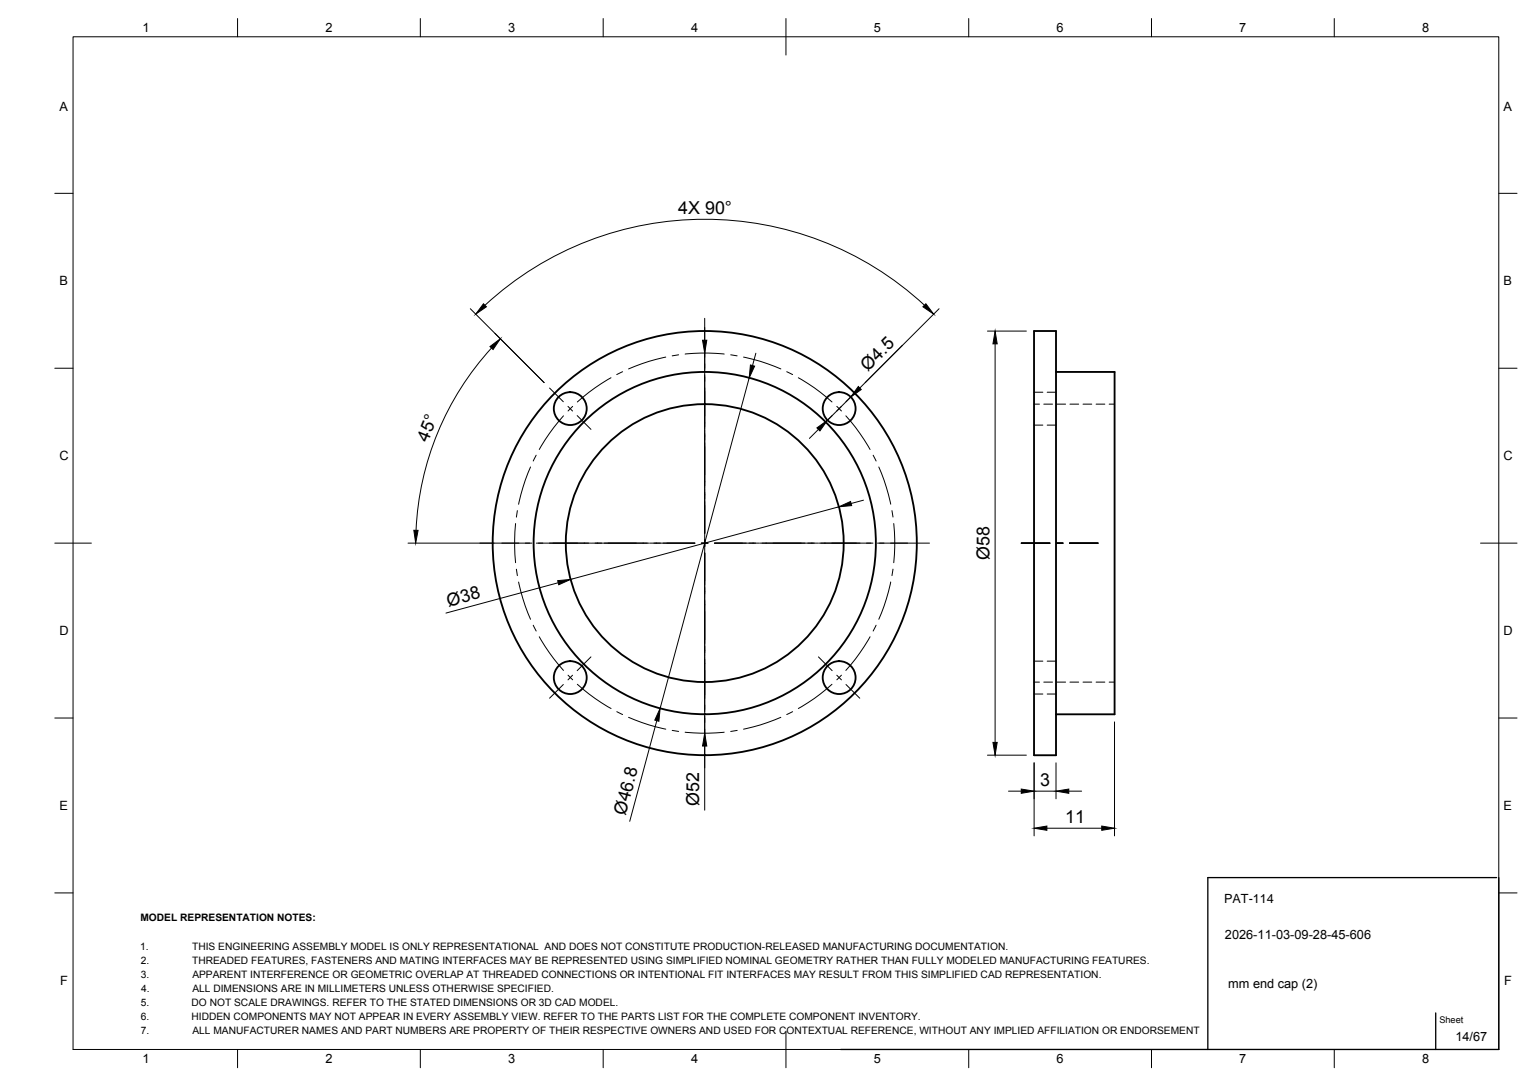
ISO-10303-21;
HEADER;
/* Generated by software containing ST-Developer
 * from STEP Tools, Inc. (www.steptools.com) 
 */

FILE_DESCRIPTION(
/* description */ ('Two-stage gear reducer in split housing'),
/* implementation_level */ '2;1');

FILE_NAME(
/* name */ 'mm end cap (2).step',
/* time_stamp */ '2026-10-28T03:22:31-07:00',
/* author */ (''),
/* organization */ (''),
/* preprocessor_version */ 'ST-DEVELOPER v20.2',
/* originating_system */ 'Autodesk Translation Framework v15.17.0.0',
/* authorisation */ '');

FILE_SCHEMA (('AUTOMOTIVE_DESIGN { 1 0 10303 214 3 1 1 }'));
ENDSEC;

DATA;
#10=MECHANICAL_DESIGN_GEOMETRIC_PRESENTATION_REPRESENTATION('',(#1243),#73366);
#1131=SHAPE_REPRESENTATION_RELATIONSHIP('SRR','None',#73618,#1187);
#1187=ADVANCED_BREP_SHAPE_REPRESENTATION('',(#1314),#73314);
#1243=STYLED_ITEM('',(#74002),#1314);
#1314=MANIFOLD_SOLID_BREP('Body1',#16131);
#1466=FACE_BOUND('',#3233,.T.);
#1467=FACE_BOUND('',#3237,.T.);
#1468=FACE_BOUND('',#3238,.T.);
#1469=FACE_BOUND('',#3239,.T.);
#1470=FACE_BOUND('',#3240,.T.);
#1471=FACE_BOUND('',#3241,.T.);
#1472=FACE_BOUND('',#3243,.T.);
#1473=FACE_BOUND('',#3244,.T.);
#1474=FACE_BOUND('',#3245,.T.);
#1475=FACE_BOUND('',#3246,.T.);
#1476=FACE_BOUND('',#3247,.T.);
#1714=PLANE('',#17275);
#1715=PLANE('',#17282);
#1716=PLANE('',#17283);
#2222=FACE_OUTER_BOUND('',#3227,.T.);
#2223=FACE_OUTER_BOUND('',#3228,.T.);
#2224=FACE_OUTER_BOUND('',#3229,.T.);
#2225=FACE_OUTER_BOUND('',#3230,.T.);
#2226=FACE_OUTER_BOUND('',#3231,.T.);
#2227=FACE_OUTER_BOUND('',#3232,.T.);
#2228=FACE_OUTER_BOUND('',#3234,.T.);
#2229=FACE_OUTER_BOUND('',#3235,.T.);
#2230=FACE_OUTER_BOUND('',#3236,.T.);
#2231=FACE_OUTER_BOUND('',#3242,.T.);
#3227=EDGE_LOOP('',(#11491,#11492,#11493,#11494));
#3228=EDGE_LOOP('',(#11495,#11496,#11497,#11498));
#3229=EDGE_LOOP('',(#11499,#11500,#11501,#11502));
#3230=EDGE_LOOP('',(#11503,#11504,#11505,#11506));
#3231=EDGE_LOOP('',(#11507,#11508,#11509,#11510));
#3232=EDGE_LOOP('',(#11511));
#3233=EDGE_LOOP('',(#11512));
#3234=EDGE_LOOP('',(#11513,#11514,#11515,#11516));
#3235=EDGE_LOOP('',(#11517,#11518,#11519,#11520));
#3236=EDGE_LOOP('',(#11521));
#3237=EDGE_LOOP('',(#11522));
#3238=EDGE_LOOP('',(#11523));
#3239=EDGE_LOOP('',(#11524));
#3240=EDGE_LOOP('',(#11525));
#3241=EDGE_LOOP('',(#11526));
#3242=EDGE_LOOP('',(#11527));
#3243=EDGE_LOOP('',(#11528));
#3244=EDGE_LOOP('',(#11529));
#3245=EDGE_LOOP('',(#11530));
#3246=EDGE_LOOP('',(#11531));
#3247=EDGE_LOOP('',(#11532));
#4332=LINE('',#23830,#5356);
#4333=LINE('',#23836,#5357);
#4334=LINE('',#23842,#5358);
#4335=LINE('',#23848,#5359);
#4336=LINE('',#23854,#5360);
#4337=LINE('',#23861,#5361);
#4338=LINE('',#23867,#5362);
#5356=VECTOR('',#19634,0.225);
#5357=VECTOR('',#19641,0.225);
#5358=VECTOR('',#19648,0.225000000000001);
#5359=VECTOR('',#19655,0.225000000000001);
#5360=VECTOR('',#19662,2.34);
#5361=VECTOR('',#19671,1.9);
#5362=VECTOR('',#19678,2.9);
#6320=CIRCLE('',#17261,0.225);
#6321=CIRCLE('',#17262,0.225);
#6322=CIRCLE('',#17264,0.225);
#6323=CIRCLE('',#17265,0.225);
#6324=CIRCLE('',#17267,0.225000000000001);
#6325=CIRCLE('',#17268,0.225000000000001);
#6326=CIRCLE('',#17270,0.225000000000001);
#6327=CIRCLE('',#17271,0.225000000000001);
#6328=CIRCLE('',#17273,2.34);
#6329=CIRCLE('',#17274,2.34);
#6330=CIRCLE('',#17276,1.9);
#6331=CIRCLE('',#17278,1.9);
#6332=CIRCLE('',#17280,2.9);
#6333=CIRCLE('',#17281,2.9);
#7152=VERTEX_POINT('',#23827);
#7153=VERTEX_POINT('',#23829);
#7154=VERTEX_POINT('',#23833);
#7155=VERTEX_POINT('',#23835);
#7156=VERTEX_POINT('',#23839);
#7157=VERTEX_POINT('',#23841);
#7158=VERTEX_POINT('',#23845);
#7159=VERTEX_POINT('',#23847);
#7160=VERTEX_POINT('',#23851);
#7161=VERTEX_POINT('',#23853);
#7162=VERTEX_POINT('',#23857);
#7163=VERTEX_POINT('',#23860);
#7164=VERTEX_POINT('',#23864);
#7165=VERTEX_POINT('',#23866);
#8799=EDGE_CURVE('',#7152,#7152,#6320,.T.);
#8800=EDGE_CURVE('',#7152,#7153,#4332,.T.);
#8801=EDGE_CURVE('',#7153,#7153,#6321,.T.);
#8802=EDGE_CURVE('',#7154,#7154,#6322,.T.);
#8803=EDGE_CURVE('',#7154,#7155,#4333,.T.);
#8804=EDGE_CURVE('',#7155,#7155,#6323,.T.);
#8805=EDGE_CURVE('',#7156,#7156,#6324,.T.);
#8806=EDGE_CURVE('',#7156,#7157,#4334,.T.);
#8807=EDGE_CURVE('',#7157,#7157,#6325,.T.);
#8808=EDGE_CURVE('',#7158,#7158,#6326,.T.);
#8809=EDGE_CURVE('',#7158,#7159,#4335,.T.);
#8810=EDGE_CURVE('',#7159,#7159,#6327,.T.);
#8811=EDGE_CURVE('',#7160,#7160,#6328,.T.);
#8812=EDGE_CURVE('',#7160,#7161,#4336,.T.);
#8813=EDGE_CURVE('',#7161,#7161,#6329,.T.);
#8814=EDGE_CURVE('',#7162,#7162,#6330,.T.);
#8815=EDGE_CURVE('',#7162,#7163,#4337,.T.);
#8816=EDGE_CURVE('',#7163,#7163,#6331,.T.);
#8817=EDGE_CURVE('',#7164,#7164,#6332,.T.);
#8818=EDGE_CURVE('',#7164,#7165,#4338,.T.);
#8819=EDGE_CURVE('',#7165,#7165,#6333,.T.);
#11491=ORIENTED_EDGE('',*,*,#8799,.F.);
#11492=ORIENTED_EDGE('',*,*,#8800,.T.);
#11493=ORIENTED_EDGE('',*,*,#8801,.F.);
#11494=ORIENTED_EDGE('',*,*,#8800,.F.);
#11495=ORIENTED_EDGE('',*,*,#8802,.F.);
#11496=ORIENTED_EDGE('',*,*,#8803,.T.);
#11497=ORIENTED_EDGE('',*,*,#8804,.F.);
#11498=ORIENTED_EDGE('',*,*,#8803,.F.);
#11499=ORIENTED_EDGE('',*,*,#8805,.F.);
#11500=ORIENTED_EDGE('',*,*,#8806,.T.);
#11501=ORIENTED_EDGE('',*,*,#8807,.F.);
#11502=ORIENTED_EDGE('',*,*,#8806,.F.);
#11503=ORIENTED_EDGE('',*,*,#8808,.F.);
#11504=ORIENTED_EDGE('',*,*,#8809,.T.);
#11505=ORIENTED_EDGE('',*,*,#8810,.F.);
#11506=ORIENTED_EDGE('',*,*,#8809,.F.);
#11507=ORIENTED_EDGE('',*,*,#8811,.F.);
#11508=ORIENTED_EDGE('',*,*,#8812,.T.);
#11509=ORIENTED_EDGE('',*,*,#8813,.F.);
#11510=ORIENTED_EDGE('',*,*,#8812,.F.);
#11511=ORIENTED_EDGE('',*,*,#8811,.T.);
#11512=ORIENTED_EDGE('',*,*,#8814,.T.);
#11513=ORIENTED_EDGE('',*,*,#8814,.F.);
#11514=ORIENTED_EDGE('',*,*,#8815,.T.);
#11515=ORIENTED_EDGE('',*,*,#8816,.T.);
#11516=ORIENTED_EDGE('',*,*,#8815,.F.);
#11517=ORIENTED_EDGE('',*,*,#8817,.F.);
#11518=ORIENTED_EDGE('',*,*,#8818,.T.);
#11519=ORIENTED_EDGE('',*,*,#8819,.T.);
#11520=ORIENTED_EDGE('',*,*,#8818,.F.);
#11521=ORIENTED_EDGE('',*,*,#8817,.T.);
#11522=ORIENTED_EDGE('',*,*,#8813,.T.);
#11523=ORIENTED_EDGE('',*,*,#8810,.T.);
#11524=ORIENTED_EDGE('',*,*,#8807,.T.);
#11525=ORIENTED_EDGE('',*,*,#8804,.T.);
#11526=ORIENTED_EDGE('',*,*,#8801,.T.);
#11527=ORIENTED_EDGE('',*,*,#8819,.F.);
#11528=ORIENTED_EDGE('',*,*,#8816,.F.);
#11529=ORIENTED_EDGE('',*,*,#8808,.T.);
#11530=ORIENTED_EDGE('',*,*,#8805,.T.);
#11531=ORIENTED_EDGE('',*,*,#8802,.T.);
#11532=ORIENTED_EDGE('',*,*,#8799,.T.);
#15015=CYLINDRICAL_SURFACE('',#17260,0.225);
#15016=CYLINDRICAL_SURFACE('',#17263,0.225);
#15017=CYLINDRICAL_SURFACE('',#17266,0.225000000000001);
#15018=CYLINDRICAL_SURFACE('',#17269,0.225000000000001);
#15019=CYLINDRICAL_SURFACE('',#17272,2.34);
#15020=CYLINDRICAL_SURFACE('',#17277,1.9);
#15021=CYLINDRICAL_SURFACE('',#17279,2.9);
#15429=ADVANCED_FACE('',(#2222),#15015,.F.);
#15430=ADVANCED_FACE('',(#2223),#15016,.F.);
#15431=ADVANCED_FACE('',(#2224),#15017,.F.);
#15432=ADVANCED_FACE('',(#2225),#15018,.F.);
#15433=ADVANCED_FACE('',(#2226),#15019,.T.);
#15434=ADVANCED_FACE('',(#2227,#1466),#1714,.T.);
#15435=ADVANCED_FACE('',(#2228),#15020,.F.);
#15436=ADVANCED_FACE('',(#2229),#15021,.T.);
#15437=ADVANCED_FACE('',(#2230,#1467,#1468,#1469,#1470,#1471),#1715,.T.);
#15438=ADVANCED_FACE('',(#2231,#1472,#1473,#1474,#1475,#1476),#1716,.F.);
#16131=CLOSED_SHELL('',(#15429,#15430,#15431,#15432,#15433,#15434,#15435,
#15436,#15437,#15438));
#17259=AXIS2_PLACEMENT_3D('',#23825,#19628,#19629);
#17260=AXIS2_PLACEMENT_3D('',#23826,#19630,#19631);
#17261=AXIS2_PLACEMENT_3D('',#23828,#19632,#19633);
#17262=AXIS2_PLACEMENT_3D('',#23831,#19635,#19636);
#17263=AXIS2_PLACEMENT_3D('',#23832,#19637,#19638);
#17264=AXIS2_PLACEMENT_3D('',#23834,#19639,#19640);
#17265=AXIS2_PLACEMENT_3D('',#23837,#19642,#19643);
#17266=AXIS2_PLACEMENT_3D('',#23838,#19644,#19645);
#17267=AXIS2_PLACEMENT_3D('',#23840,#19646,#19647);
#17268=AXIS2_PLACEMENT_3D('',#23843,#19649,#19650);
#17269=AXIS2_PLACEMENT_3D('',#23844,#19651,#19652);
#17270=AXIS2_PLACEMENT_3D('',#23846,#19653,#19654);
#17271=AXIS2_PLACEMENT_3D('',#23849,#19656,#19657);
#17272=AXIS2_PLACEMENT_3D('',#23850,#19658,#19659);
#17273=AXIS2_PLACEMENT_3D('',#23852,#19660,#19661);
#17274=AXIS2_PLACEMENT_3D('',#23855,#19663,#19664);
#17275=AXIS2_PLACEMENT_3D('',#23856,#19665,#19666);
#17276=AXIS2_PLACEMENT_3D('',#23858,#19667,#19668);
#17277=AXIS2_PLACEMENT_3D('',#23859,#19669,#19670);
#17278=AXIS2_PLACEMENT_3D('',#23862,#19672,#19673);
#17279=AXIS2_PLACEMENT_3D('',#23863,#19674,#19675);
#17280=AXIS2_PLACEMENT_3D('',#23865,#19676,#19677);
#17281=AXIS2_PLACEMENT_3D('',#23868,#19679,#19680);
#17282=AXIS2_PLACEMENT_3D('',#23869,#19681,#19682);
#17283=AXIS2_PLACEMENT_3D('',#23870,#19683,#19684);
#19628=DIRECTION('axis',(0.,0.,1.));
#19629=DIRECTION('refdir',(1.,0.,0.));
#19630=DIRECTION('center_axis',(0.,1.,0.));
#19631=DIRECTION('ref_axis',(1.,0.,0.));
#19632=DIRECTION('center_axis',(0.,1.,0.));
#19633=DIRECTION('ref_axis',(1.,0.,0.));
#19634=DIRECTION('',(0.,1.,0.));
#19635=DIRECTION('center_axis',(0.,-1.,0.));
#19636=DIRECTION('ref_axis',(1.,0.,0.));
#19637=DIRECTION('center_axis',(0.,1.,0.));
#19638=DIRECTION('ref_axis',(1.,0.,0.));
#19639=DIRECTION('center_axis',(0.,1.,0.));
#19640=DIRECTION('ref_axis',(1.,0.,0.));
#19641=DIRECTION('',(0.,1.,0.));
#19642=DIRECTION('center_axis',(0.,-1.,0.));
#19643=DIRECTION('ref_axis',(1.,0.,0.));
#19644=DIRECTION('center_axis',(0.,1.,0.));
#19645=DIRECTION('ref_axis',(1.,0.,0.));
#19646=DIRECTION('center_axis',(0.,1.,0.));
#19647=DIRECTION('ref_axis',(1.,0.,0.));
#19648=DIRECTION('',(0.,1.,0.));
#19649=DIRECTION('center_axis',(0.,-1.,0.));
#19650=DIRECTION('ref_axis',(1.,0.,0.));
#19651=DIRECTION('center_axis',(0.,1.,0.));
#19652=DIRECTION('ref_axis',(1.,0.,0.));
#19653=DIRECTION('center_axis',(0.,1.,0.));
#19654=DIRECTION('ref_axis',(1.,0.,0.));
#19655=DIRECTION('',(0.,1.,0.));
#19656=DIRECTION('center_axis',(0.,-1.,0.));
#19657=DIRECTION('ref_axis',(1.,0.,0.));
#19658=DIRECTION('center_axis',(0.,1.,0.));
#19659=DIRECTION('ref_axis',(1.,0.,0.));
#19660=DIRECTION('center_axis',(0.,1.,0.));
#19661=DIRECTION('ref_axis',(1.,0.,0.));
#19662=DIRECTION('',(0.,-1.,0.));
#19663=DIRECTION('center_axis',(0.,-1.,0.));
#19664=DIRECTION('ref_axis',(1.,0.,0.));
#19665=DIRECTION('center_axis',(0.,1.,0.));
#19666=DIRECTION('ref_axis',(1.,0.,0.));
#19667=DIRECTION('center_axis',(0.,-1.,0.));
#19668=DIRECTION('ref_axis',(1.,0.,0.));
#19669=DIRECTION('center_axis',(0.,1.,0.));
#19670=DIRECTION('ref_axis',(1.,0.,0.));
#19671=DIRECTION('',(0.,-1.,0.));
#19672=DIRECTION('center_axis',(0.,-1.,0.));
#19673=DIRECTION('ref_axis',(1.,0.,0.));
#19674=DIRECTION('center_axis',(0.,1.,0.));
#19675=DIRECTION('ref_axis',(1.,0.,0.));
#19676=DIRECTION('center_axis',(0.,1.,0.));
#19677=DIRECTION('ref_axis',(1.,0.,0.));
#19678=DIRECTION('',(0.,-1.,0.));
#19679=DIRECTION('center_axis',(0.,1.,0.));
#19680=DIRECTION('ref_axis',(1.,0.,0.));
#19681=DIRECTION('center_axis',(0.,1.,0.));
#19682=DIRECTION('ref_axis',(1.,0.,0.));
#19683=DIRECTION('center_axis',(0.,1.,0.));
#19684=DIRECTION('ref_axis',(1.,0.,0.));
#23825=CARTESIAN_POINT('',(0.,0.,0.));
#23826=CARTESIAN_POINT('Origin',(4.16152236891498,-7.9,8.16152236891498));
#23827=CARTESIAN_POINT('',(3.93652236891498,-7.8,8.16152236891498));
#23828=CARTESIAN_POINT('Origin',(4.16152236891498,-7.8,8.16152236891498));
#23829=CARTESIAN_POINT('',(3.93652236891498,-7.5,8.16152236891498));
#23830=CARTESIAN_POINT('',(3.93652236891498,-7.9,8.16152236891498));
#23831=CARTESIAN_POINT('Origin',(4.16152236891498,-7.5,8.16152236891498));
#23832=CARTESIAN_POINT('Origin',(4.16152236891498,-7.9,11.838477631085));
#23833=CARTESIAN_POINT('',(3.93652236891498,-7.8,11.838477631085));
#23834=CARTESIAN_POINT('Origin',(4.16152236891498,-7.8,11.838477631085));
#23835=CARTESIAN_POINT('',(3.93652236891498,-7.5,11.838477631085));
#23836=CARTESIAN_POINT('',(3.93652236891498,-7.9,11.838477631085));
#23837=CARTESIAN_POINT('Origin',(4.16152236891498,-7.5,11.838477631085));
#23838=CARTESIAN_POINT('Origin',(7.83847763108502,-7.9,11.838477631085));
#23839=CARTESIAN_POINT('',(7.61347763108502,-7.8,11.838477631085));
#23840=CARTESIAN_POINT('Origin',(7.83847763108502,-7.8,11.838477631085));
#23841=CARTESIAN_POINT('',(7.61347763108502,-7.5,11.838477631085));
#23842=CARTESIAN_POINT('',(7.61347763108502,-7.9,11.838477631085));
#23843=CARTESIAN_POINT('Origin',(7.83847763108502,-7.5,11.838477631085));
#23844=CARTESIAN_POINT('Origin',(7.83847763108502,-7.9,8.16152236891498));
#23845=CARTESIAN_POINT('',(7.61347763108502,-7.8,8.16152236891498));
#23846=CARTESIAN_POINT('Origin',(7.83847763108502,-7.8,8.16152236891498));
#23847=CARTESIAN_POINT('',(7.61347763108502,-7.5,8.16152236891498));
#23848=CARTESIAN_POINT('',(7.61347763108502,-7.9,8.16152236891498));
#23849=CARTESIAN_POINT('Origin',(7.83847763108502,-7.5,8.16152236891498));
#23850=CARTESIAN_POINT('Origin',(6.,-7.5,10.));
#23851=CARTESIAN_POINT('',(3.66,-6.7,10.));
#23852=CARTESIAN_POINT('Origin',(6.,-6.7,10.));
#23853=CARTESIAN_POINT('',(3.66,-7.5,10.));
#23854=CARTESIAN_POINT('',(3.66,-7.5,10.));
#23855=CARTESIAN_POINT('Origin',(6.,-7.5,10.));
#23856=CARTESIAN_POINT('Origin',(6.,-6.7,10.));
#23857=CARTESIAN_POINT('',(4.1,-6.7,10.));
#23858=CARTESIAN_POINT('Origin',(6.,-6.7,10.));
#23859=CARTESIAN_POINT('Origin',(6.,-7.8,10.));
#23860=CARTESIAN_POINT('',(4.1,-7.8,10.));
#23861=CARTESIAN_POINT('',(4.1,-7.8,10.));
#23862=CARTESIAN_POINT('Origin',(6.,-7.8,10.));
#23863=CARTESIAN_POINT('Origin',(6.,-7.8,10.));
#23864=CARTESIAN_POINT('',(3.1,-7.5,10.));
#23865=CARTESIAN_POINT('Origin',(6.,-7.5,10.));
#23866=CARTESIAN_POINT('',(3.1,-7.8,10.));
#23867=CARTESIAN_POINT('',(3.1,-7.8,10.));
#23868=CARTESIAN_POINT('Origin',(6.,-7.8,10.));
#23869=CARTESIAN_POINT('Origin',(6.,-7.5,10.));
#23870=CARTESIAN_POINT('Origin',(6.,-7.8,10.));
#73250=UNCERTAINTY_MEASURE_WITH_UNIT(LENGTH_MEASURE(0.001),#73367,
'DISTANCE_ACCURACY_VALUE',
'Maximum model space distance between geometric entities at asserted c
onnectivities');
#73302=UNCERTAINTY_MEASURE_WITH_UNIT(LENGTH_MEASURE(0.001),#73367,
'DISTANCE_ACCURACY_VALUE',
'Maximum model space distance between geometric entities at asserted c
onnectivities');
#73314=(
GEOMETRIC_REPRESENTATION_CONTEXT(3)
GLOBAL_UNCERTAINTY_ASSIGNED_CONTEXT((#73250))
GLOBAL_UNIT_ASSIGNED_CONTEXT((#73367,#73369,#73370))
REPRESENTATION_CONTEXT('','3D')
);
#73366=(
GEOMETRIC_REPRESENTATION_CONTEXT(3)
GLOBAL_UNCERTAINTY_ASSIGNED_CONTEXT((#73302))
GLOBAL_UNIT_ASSIGNED_CONTEXT((#73367,#73369,#73370))
REPRESENTATION_CONTEXT('','3D')
);
#73367=(
LENGTH_UNIT()
NAMED_UNIT(*)
SI_UNIT(.CENTI.,.METRE.)
);
#73369=(
NAMED_UNIT(*)
PLANE_ANGLE_UNIT()
SI_UNIT($,.RADIAN.)
);
#73370=(
NAMED_UNIT(*)
SI_UNIT($,.STERADIAN.)
SOLID_ANGLE_UNIT()
);
#73382=SHAPE_DEFINITION_REPRESENTATION(#73445,#73618);
#73445=PRODUCT_DEFINITION_SHAPE('',$,#73682);
#73618=SHAPE_REPRESENTATION('',(#17259),#73314);
#73670=PRODUCT_DEFINITION_CONTEXT('part definition',#73861,'design');
#73682=PRODUCT_DEFINITION('mm end cap (2)','mm end cap (2)',#73745,#73670);
#73745=PRODUCT_DEFINITION_FORMATION('',$,#73874);
#73861=APPLICATION_CONTEXT(
'Core Data for Automotive Mechanical Design Process');
#73862=PRODUCT_CONTEXT('part definition',#73861,'mechanical');
#73874=PRODUCT('mm end cap (2)','mm end cap (2)','mm end cap (2)',(#73862));
#73996=COLOUR_RGB('Off White',0.89,0.88,0.83);
#73997=FILL_AREA_STYLE_COLOUR('',#73996);
#73998=FILL_AREA_STYLE('',(#73997));
#73999=SURFACE_STYLE_FILL_AREA(#73998);
#74000=SURFACE_SIDE_STYLE('',(#73999));
#74001=SURFACE_STYLE_USAGE(.BOTH.,#74000);
#74002=PRESENTATION_STYLE_ASSIGNMENT((#74001));
ENDSEC;
END-ISO-10303-21;
